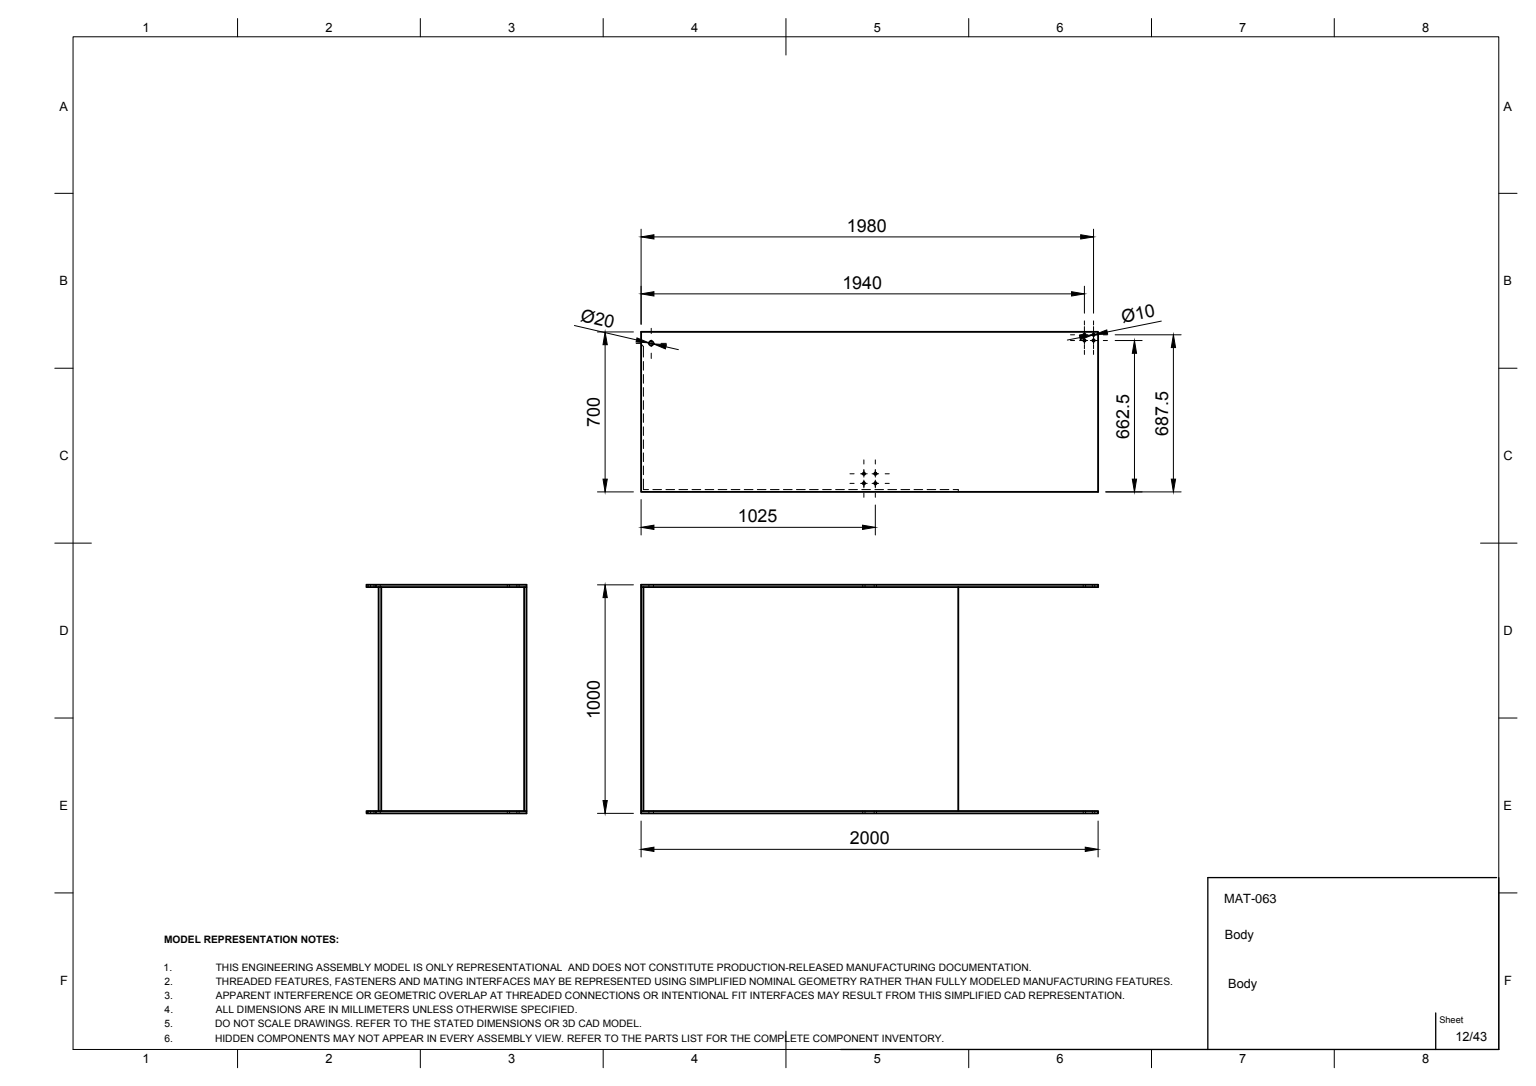
ISO-10303-21;
HEADER;
/* Generated by software containing ST-Developer
 * from STEP Tools, Inc. (www.steptools.com) 
 */

FILE_DESCRIPTION(
/* description */ (''),
/* implementation_level */ '2;1');

FILE_NAME(
/* name */ 'Body.step',
/* time_stamp */ '2026-10-24T09:43:01-07:00',
/* author */ (''),
/* organization */ (''),
/* preprocessor_version */ 'ST-DEVELOPER v20.2',
/* originating_system */ 'Autodesk Translation Framework v15.15.0.0',
/* authorisation */ '');

FILE_SCHEMA (('AUTOMOTIVE_DESIGN { 1 0 10303 214 3 1 1 }'));
ENDSEC;

DATA;
#10=MECHANICAL_DESIGN_GEOMETRIC_PRESENTATION_REPRESENTATION('',(#289),#11112);
#223=SHAPE_REPRESENTATION_RELATIONSHIP('SRR','None',#11247,#256);
#256=ADVANCED_BREP_SHAPE_REPRESENTATION('',(#322),#11092);
#289=STYLED_ITEM('',(#11426),#322);
#322=MANIFOLD_SOLID_BREP('Body',#6026);
#417=FACE_BOUND('',#1348,.T.);
#418=FACE_BOUND('',#1349,.T.);
#419=FACE_BOUND('',#1350,.T.);
#420=FACE_BOUND('',#1351,.T.);
#421=FACE_BOUND('',#1352,.T.);
#422=FACE_BOUND('',#1353,.T.);
#423=FACE_BOUND('',#1354,.T.);
#424=FACE_BOUND('',#1355,.T.);
#425=FACE_BOUND('',#1356,.T.);
#426=FACE_BOUND('',#1358,.T.);
#427=FACE_BOUND('',#1359,.T.);
#428=FACE_BOUND('',#1360,.T.);
#429=FACE_BOUND('',#1361,.T.);
#430=FACE_BOUND('',#1362,.T.);
#431=FACE_BOUND('',#1363,.T.);
#432=FACE_BOUND('',#1364,.T.);
#433=FACE_BOUND('',#1365,.T.);
#434=FACE_BOUND('',#1366,.T.);
#435=FACE_BOUND('',#1385,.T.);
#436=FACE_BOUND('',#1386,.T.);
#437=FACE_BOUND('',#1387,.T.);
#438=FACE_BOUND('',#1388,.T.);
#439=FACE_BOUND('',#1389,.T.);
#440=FACE_BOUND('',#1390,.T.);
#441=FACE_BOUND('',#1391,.T.);
#442=FACE_BOUND('',#1392,.T.);
#443=FACE_BOUND('',#1393,.T.);
#444=FACE_BOUND('',#1395,.T.);
#445=FACE_BOUND('',#1396,.T.);
#446=FACE_BOUND('',#1397,.T.);
#447=FACE_BOUND('',#1398,.T.);
#448=FACE_BOUND('',#1399,.T.);
#449=FACE_BOUND('',#1400,.T.);
#450=FACE_BOUND('',#1401,.T.);
#451=FACE_BOUND('',#1402,.T.);
#452=FACE_BOUND('',#1403,.T.);
#592=PLANE('',#6965);
#593=PLANE('',#6974);
#594=PLANE('',#6991);
#595=PLANE('',#6992);
#596=PLANE('',#6993);
#597=PLANE('',#6994);
#598=PLANE('',#6995);
#599=PLANE('',#6996);
#600=PLANE('',#6997);
#601=PLANE('',#6998);
#602=PLANE('',#6999);
#603=PLANE('',#7000);
#604=PLANE('',#7010);
#605=PLANE('',#7020);
#904=FACE_OUTER_BOUND('',#1346,.T.);
#905=FACE_OUTER_BOUND('',#1347,.T.);
#906=FACE_OUTER_BOUND('',#1357,.T.);
#907=FACE_OUTER_BOUND('',#1367,.T.);
#908=FACE_OUTER_BOUND('',#1368,.T.);
#909=FACE_OUTER_BOUND('',#1369,.T.);
#910=FACE_OUTER_BOUND('',#1370,.T.);
#911=FACE_OUTER_BOUND('',#1371,.T.);
#912=FACE_OUTER_BOUND('',#1372,.T.);
#913=FACE_OUTER_BOUND('',#1373,.T.);
#914=FACE_OUTER_BOUND('',#1374,.T.);
#915=FACE_OUTER_BOUND('',#1375,.T.);
#916=FACE_OUTER_BOUND('',#1376,.T.);
#917=FACE_OUTER_BOUND('',#1377,.T.);
#918=FACE_OUTER_BOUND('',#1378,.T.);
#919=FACE_OUTER_BOUND('',#1379,.T.);
#920=FACE_OUTER_BOUND('',#1380,.T.);
#921=FACE_OUTER_BOUND('',#1381,.T.);
#922=FACE_OUTER_BOUND('',#1382,.T.);
#923=FACE_OUTER_BOUND('',#1383,.T.);
#924=FACE_OUTER_BOUND('',#1384,.T.);
#925=FACE_OUTER_BOUND('',#1394,.T.);
#926=FACE_OUTER_BOUND('',#1404,.T.);
#927=FACE_OUTER_BOUND('',#1405,.T.);
#928=FACE_OUTER_BOUND('',#1406,.T.);
#929=FACE_OUTER_BOUND('',#1407,.T.);
#930=FACE_OUTER_BOUND('',#1408,.T.);
#931=FACE_OUTER_BOUND('',#1409,.T.);
#932=FACE_OUTER_BOUND('',#1410,.T.);
#933=FACE_OUTER_BOUND('',#1411,.T.);
#934=FACE_OUTER_BOUND('',#1412,.T.);
#935=FACE_OUTER_BOUND('',#1413,.T.);
#1346=EDGE_LOOP('',(#4915,#4916,#4917,#4918));
#1347=EDGE_LOOP('',(#4919,#4920,#4921,#4922));
#1348=EDGE_LOOP('',(#4923));
#1349=EDGE_LOOP('',(#4924));
#1350=EDGE_LOOP('',(#4925));
#1351=EDGE_LOOP('',(#4926));
#1352=EDGE_LOOP('',(#4927));
#1353=EDGE_LOOP('',(#4928));
#1354=EDGE_LOOP('',(#4929));
#1355=EDGE_LOOP('',(#4930));
#1356=EDGE_LOOP('',(#4931));
#1357=EDGE_LOOP('',(#4932,#4933,#4934,#4935,#4936,#4937,#4938,#4939));
#1358=EDGE_LOOP('',(#4940));
#1359=EDGE_LOOP('',(#4941));
#1360=EDGE_LOOP('',(#4942));
#1361=EDGE_LOOP('',(#4943));
#1362=EDGE_LOOP('',(#4944));
#1363=EDGE_LOOP('',(#4945));
#1364=EDGE_LOOP('',(#4946));
#1365=EDGE_LOOP('',(#4947));
#1366=EDGE_LOOP('',(#4948));
#1367=EDGE_LOOP('',(#4949,#4950,#4951,#4952));
#1368=EDGE_LOOP('',(#4953,#4954,#4955,#4956));
#1369=EDGE_LOOP('',(#4957,#4958,#4959,#4960));
#1370=EDGE_LOOP('',(#4961,#4962,#4963,#4964));
#1371=EDGE_LOOP('',(#4965,#4966,#4967,#4968));
#1372=EDGE_LOOP('',(#4969,#4970,#4971,#4972));
#1373=EDGE_LOOP('',(#4973,#4974,#4975,#4976));
#1374=EDGE_LOOP('',(#4977,#4978,#4979,#4980));
#1375=EDGE_LOOP('',(#4981,#4982,#4983,#4984,#4985,#4986,#4987,#4988));
#1376=EDGE_LOOP('',(#4989,#4990,#4991,#4992));
#1377=EDGE_LOOP('',(#4993,#4994,#4995,#4996));
#1378=EDGE_LOOP('',(#4997,#4998,#4999,#5000,#5001,#5002,#5003,#5004));
#1379=EDGE_LOOP('',(#5005,#5006,#5007,#5008));
#1380=EDGE_LOOP('',(#5009,#5010,#5011,#5012));
#1381=EDGE_LOOP('',(#5013,#5014,#5015,#5016));
#1382=EDGE_LOOP('',(#5017,#5018,#5019,#5020));
#1383=EDGE_LOOP('',(#5021,#5022,#5023,#5024));
#1384=EDGE_LOOP('',(#5025,#5026,#5027,#5028,#5029,#5030,#5031,#5032));
#1385=EDGE_LOOP('',(#5033));
#1386=EDGE_LOOP('',(#5034));
#1387=EDGE_LOOP('',(#5035));
#1388=EDGE_LOOP('',(#5036));
#1389=EDGE_LOOP('',(#5037));
#1390=EDGE_LOOP('',(#5038));
#1391=EDGE_LOOP('',(#5039));
#1392=EDGE_LOOP('',(#5040));
#1393=EDGE_LOOP('',(#5041));
#1394=EDGE_LOOP('',(#5042,#5043,#5044,#5045));
#1395=EDGE_LOOP('',(#5046));
#1396=EDGE_LOOP('',(#5047));
#1397=EDGE_LOOP('',(#5048));
#1398=EDGE_LOOP('',(#5049));
#1399=EDGE_LOOP('',(#5050));
#1400=EDGE_LOOP('',(#5051));
#1401=EDGE_LOOP('',(#5052));
#1402=EDGE_LOOP('',(#5053));
#1403=EDGE_LOOP('',(#5054));
#1404=EDGE_LOOP('',(#5055,#5056,#5057,#5058));
#1405=EDGE_LOOP('',(#5059,#5060,#5061,#5062));
#1406=EDGE_LOOP('',(#5063,#5064,#5065,#5066));
#1407=EDGE_LOOP('',(#5067,#5068,#5069,#5070));
#1408=EDGE_LOOP('',(#5071,#5072,#5073,#5074));
#1409=EDGE_LOOP('',(#5075,#5076,#5077,#5078));
#1410=EDGE_LOOP('',(#5079,#5080,#5081,#5082));
#1411=EDGE_LOOP('',(#5083,#5084,#5085,#5086));
#1412=EDGE_LOOP('',(#5087,#5088,#5089,#5090));
#1413=EDGE_LOOP('',(#5091,#5092,#5093,#5094));
#1741=LINE('',#10369,#2100);
#1742=LINE('',#10374,#2101);
#1743=LINE('',#10376,#2102);
#1744=LINE('',#10378,#2103);
#1745=LINE('',#10379,#2104);
#1746=LINE('',#10399,#2105);
#1747=LINE('',#10401,#2106);
#1748=LINE('',#10403,#2107);
#1749=LINE('',#10405,#2108);
#1750=LINE('',#10407,#2109);
#1751=LINE('',#10409,#2110);
#1752=LINE('',#10411,#2111);
#1753=LINE('',#10412,#2112);
#1754=LINE('',#10430,#2113);
#1755=LINE('',#10432,#2114);
#1756=LINE('',#10434,#2115);
#1757=LINE('',#10436,#2116);
#1758=LINE('',#10438,#2117);
#1759=LINE('',#10440,#2118);
#1760=LINE('',#10442,#2119);
#1761=LINE('',#10444,#2120);
#1762=LINE('',#10448,#2121);
#1763=LINE('',#10450,#2122);
#1764=LINE('',#10452,#2123);
#1765=LINE('',#10453,#2124);
#1766=LINE('',#10454,#2125);
#1767=LINE('',#10455,#2126);
#1768=LINE('',#10457,#2127);
#1769=LINE('',#10459,#2128);
#1770=LINE('',#10462,#2129);
#1771=LINE('',#10464,#2130);
#1772=LINE('',#10466,#2131);
#1773=LINE('',#10467,#2132);
#1774=LINE('',#10470,#2133);
#1775=LINE('',#10471,#2134);
#1776=LINE('',#10474,#2135);
#1777=LINE('',#10475,#2136);
#1778=LINE('',#10478,#2137);
#1779=LINE('',#10479,#2138);
#1780=LINE('',#10481,#2139);
#1781=LINE('',#10485,#2140);
#1782=LINE('',#10486,#2141);
#1783=LINE('',#10487,#2142);
#1784=LINE('',#10489,#2143);
#1785=LINE('',#10509,#2144);
#1786=LINE('',#10530,#2145);
#1787=LINE('',#10532,#2146);
#1788=LINE('',#10534,#2147);
#1789=LINE('',#10536,#2148);
#1790=LINE('',#10538,#2149);
#1791=LINE('',#10540,#2150);
#1792=LINE('',#10542,#2151);
#1793=LINE('',#10544,#2152);
#1794=LINE('',#10546,#2153);
#2100=VECTOR('',#8557,0.01);
#2101=VECTOR('',#8562,0.01);
#2102=VECTOR('',#8563,0.01);
#2103=VECTOR('',#8564,0.01);
#2104=VECTOR('',#8565,0.01);
#2105=VECTOR('',#8584,0.01);
#2106=VECTOR('',#8585,0.01);
#2107=VECTOR('',#8586,0.01);
#2108=VECTOR('',#8587,0.01);
#2109=VECTOR('',#8588,0.01);
#2110=VECTOR('',#8589,0.01);
#2111=VECTOR('',#8590,0.01);
#2112=VECTOR('',#8591,0.01);
#2113=VECTOR('',#8610,0.00499999999997557);
#2114=VECTOR('',#8613,0.00499999999997558);
#2115=VECTOR('',#8616,0.00500000000000013);
#2116=VECTOR('',#8619,0.005);
#2117=VECTOR('',#8622,0.005);
#2118=VECTOR('',#8625,0.00500000000000013);
#2119=VECTOR('',#8628,0.00499999999997557);
#2120=VECTOR('',#8631,0.00499999999997558);
#2121=VECTOR('',#8634,0.01);
#2122=VECTOR('',#8635,0.01);
#2123=VECTOR('',#8636,0.01);
#2124=VECTOR('',#8637,0.01);
#2125=VECTOR('',#8638,0.01);
#2126=VECTOR('',#8639,0.01);
#2127=VECTOR('',#8642,0.01);
#2128=VECTOR('',#8645,0.01);
#2129=VECTOR('',#8648,0.01);
#2130=VECTOR('',#8649,0.01);
#2131=VECTOR('',#8650,0.01);
#2132=VECTOR('',#8651,0.01);
#2133=VECTOR('',#8654,0.01);
#2134=VECTOR('',#8655,0.01);
#2135=VECTOR('',#8658,0.01);
#2136=VECTOR('',#8659,0.01);
#2137=VECTOR('',#8662,0.01);
#2138=VECTOR('',#8663,0.01);
#2139=VECTOR('',#8666,0.01);
#2140=VECTOR('',#8669,0.01);
#2141=VECTOR('',#8670,0.01);
#2142=VECTOR('',#8671,0.01);
#2143=VECTOR('',#8674,0.01);
#2144=VECTOR('',#8695,0.01);
#2145=VECTOR('',#8718,0.005);
#2146=VECTOR('',#8721,0.005);
#2147=VECTOR('',#8724,0.00500000000000013);
#2148=VECTOR('',#8727,0.005);
#2149=VECTOR('',#8730,0.005);
#2150=VECTOR('',#8733,0.00500000000000013);
#2151=VECTOR('',#8736,0.005);
#2152=VECTOR('',#8739,0.005);
#2153=VECTOR('',#8742,0.01);
#2574=CIRCLE('',#6963,0.01);
#2575=CIRCLE('',#6964,0.01);
#2576=CIRCLE('',#6966,0.00499999999997558);
#2577=CIRCLE('',#6967,0.00499999999997557);
#2578=CIRCLE('',#6968,0.00500000000000013);
#2579=CIRCLE('',#6969,0.005);
#2580=CIRCLE('',#6970,0.005);
#2581=CIRCLE('',#6971,0.00500000000000013);
#2582=CIRCLE('',#6972,0.00499999999997558);
#2583=CIRCLE('',#6973,0.00499999999997557);
#2584=CIRCLE('',#6975,0.00499999999997558);
#2585=CIRCLE('',#6976,0.00499999999997557);
#2586=CIRCLE('',#6977,0.00500000000000013);
#2587=CIRCLE('',#6978,0.005);
#2588=CIRCLE('',#6979,0.005);
#2589=CIRCLE('',#6980,0.00500000000000013);
#2590=CIRCLE('',#6981,0.00499999999997558);
#2591=CIRCLE('',#6982,0.00499999999997557);
#2592=CIRCLE('',#7001,0.01);
#2593=CIRCLE('',#7002,0.005);
#2594=CIRCLE('',#7003,0.005);
#2595=CIRCLE('',#7004,0.00500000000000013);
#2596=CIRCLE('',#7005,0.005);
#2597=CIRCLE('',#7006,0.005);
#2598=CIRCLE('',#7007,0.00500000000000013);
#2599=CIRCLE('',#7008,0.005);
#2600=CIRCLE('',#7009,0.005);
#2601=CIRCLE('',#7011,0.01);
#2602=CIRCLE('',#7012,0.005);
#2603=CIRCLE('',#7013,0.005);
#2604=CIRCLE('',#7014,0.00500000000000013);
#2605=CIRCLE('',#7015,0.005);
#2606=CIRCLE('',#7016,0.005);
#2607=CIRCLE('',#7017,0.00500000000000013);
#2608=CIRCLE('',#7018,0.005);
#2609=CIRCLE('',#7019,0.005);
#2984=VERTEX_POINT('',#10366);
#2985=VERTEX_POINT('',#10368);
#2986=VERTEX_POINT('',#10372);
#2987=VERTEX_POINT('',#10373);
#2988=VERTEX_POINT('',#10375);
#2989=VERTEX_POINT('',#10377);
#2990=VERTEX_POINT('',#10380);
#2991=VERTEX_POINT('',#10382);
#2992=VERTEX_POINT('',#10384);
#2993=VERTEX_POINT('',#10386);
#2994=VERTEX_POINT('',#10388);
#2995=VERTEX_POINT('',#10390);
#2996=VERTEX_POINT('',#10392);
#2997=VERTEX_POINT('',#10394);
#2998=VERTEX_POINT('',#10397);
#2999=VERTEX_POINT('',#10398);
#3000=VERTEX_POINT('',#10400);
#3001=VERTEX_POINT('',#10402);
#3002=VERTEX_POINT('',#10404);
#3003=VERTEX_POINT('',#10406);
#3004=VERTEX_POINT('',#10408);
#3005=VERTEX_POINT('',#10410);
#3006=VERTEX_POINT('',#10413);
#3007=VERTEX_POINT('',#10415);
#3008=VERTEX_POINT('',#10417);
#3009=VERTEX_POINT('',#10419);
#3010=VERTEX_POINT('',#10421);
#3011=VERTEX_POINT('',#10423);
#3012=VERTEX_POINT('',#10425);
#3013=VERTEX_POINT('',#10427);
#3014=VERTEX_POINT('',#10446);
#3015=VERTEX_POINT('',#10447);
#3016=VERTEX_POINT('',#10449);
#3017=VERTEX_POINT('',#10451);
#3018=VERTEX_POINT('',#10461);
#3019=VERTEX_POINT('',#10463);
#3020=VERTEX_POINT('',#10465);
#3021=VERTEX_POINT('',#10469);
#3022=VERTEX_POINT('',#10473);
#3023=VERTEX_POINT('',#10477);
#3024=VERTEX_POINT('',#10483);
#3025=VERTEX_POINT('',#10484);
#3026=VERTEX_POINT('',#10490);
#3027=VERTEX_POINT('',#10492);
#3028=VERTEX_POINT('',#10494);
#3029=VERTEX_POINT('',#10496);
#3030=VERTEX_POINT('',#10498);
#3031=VERTEX_POINT('',#10500);
#3032=VERTEX_POINT('',#10502);
#3033=VERTEX_POINT('',#10504);
#3034=VERTEX_POINT('',#10506);
#3035=VERTEX_POINT('',#10510);
#3036=VERTEX_POINT('',#10512);
#3037=VERTEX_POINT('',#10514);
#3038=VERTEX_POINT('',#10516);
#3039=VERTEX_POINT('',#10518);
#3040=VERTEX_POINT('',#10520);
#3041=VERTEX_POINT('',#10522);
#3042=VERTEX_POINT('',#10524);
#3043=VERTEX_POINT('',#10526);
#3661=EDGE_CURVE('',#2984,#2984,#2574,.T.);
#3662=EDGE_CURVE('',#2984,#2985,#1741,.T.);
#3663=EDGE_CURVE('',#2985,#2985,#2575,.F.);
#3664=EDGE_CURVE('',#2986,#2987,#1742,.T.);
#3665=EDGE_CURVE('',#2988,#2986,#1743,.T.);
#3666=EDGE_CURVE('',#2989,#2988,#1744,.T.);
#3667=EDGE_CURVE('',#2987,#2989,#1745,.T.);
#3668=EDGE_CURVE('',#2990,#2990,#2576,.T.);
#3669=EDGE_CURVE('',#2991,#2991,#2577,.T.);
#3670=EDGE_CURVE('',#2992,#2992,#2578,.F.);
#3671=EDGE_CURVE('',#2993,#2993,#2579,.F.);
#3672=EDGE_CURVE('',#2994,#2994,#2580,.F.);
#3673=EDGE_CURVE('',#2995,#2995,#2581,.F.);
#3674=EDGE_CURVE('',#2996,#2996,#2582,.T.);
#3675=EDGE_CURVE('',#2997,#2997,#2583,.T.);
#3676=EDGE_CURVE('',#2998,#2999,#1746,.T.);
#3677=EDGE_CURVE('',#2999,#3000,#1747,.T.);
#3678=EDGE_CURVE('',#3000,#3001,#1748,.T.);
#3679=EDGE_CURVE('',#3001,#3002,#1749,.T.);
#3680=EDGE_CURVE('',#3002,#3003,#1750,.T.);
#3681=EDGE_CURVE('',#3003,#3004,#1751,.T.);
#3682=EDGE_CURVE('',#3004,#3005,#1752,.T.);
#3683=EDGE_CURVE('',#3005,#2998,#1753,.T.);
#3684=EDGE_CURVE('',#3006,#3006,#2584,.T.);
#3685=EDGE_CURVE('',#3007,#3007,#2585,.T.);
#3686=EDGE_CURVE('',#3008,#3008,#2586,.F.);
#3687=EDGE_CURVE('',#3009,#3009,#2587,.F.);
#3688=EDGE_CURVE('',#3010,#3010,#2588,.F.);
#3689=EDGE_CURVE('',#3011,#3011,#2589,.F.);
#3690=EDGE_CURVE('',#3012,#3012,#2590,.T.);
#3691=EDGE_CURVE('',#3013,#3013,#2591,.T.);
#3692=EDGE_CURVE('',#3013,#2997,#1754,.T.);
#3693=EDGE_CURVE('',#3006,#2996,#1755,.T.);
#3694=EDGE_CURVE('',#2995,#3011,#1756,.T.);
#3695=EDGE_CURVE('',#2994,#3010,#1757,.T.);
#3696=EDGE_CURVE('',#2993,#3009,#1758,.T.);
#3697=EDGE_CURVE('',#2992,#3008,#1759,.T.);
#3698=EDGE_CURVE('',#3007,#2991,#1760,.T.);
#3699=EDGE_CURVE('',#3012,#2990,#1761,.T.);
#3700=EDGE_CURVE('',#3014,#3015,#1762,.T.);
#3701=EDGE_CURVE('',#3016,#3014,#1763,.T.);
#3702=EDGE_CURVE('',#3017,#3016,#1764,.T.);
#3703=EDGE_CURVE('',#3001,#3017,#1765,.T.);
#3704=EDGE_CURVE('',#2988,#3000,#1766,.T.);
#3705=EDGE_CURVE('',#3015,#2986,#1767,.T.);
#3706=EDGE_CURVE('',#2989,#2999,#1768,.T.);
#3707=EDGE_CURVE('',#2987,#2998,#1769,.T.);
#3708=EDGE_CURVE('',#3018,#3005,#1770,.T.);
#3709=EDGE_CURVE('',#3019,#3018,#1771,.T.);
#3710=EDGE_CURVE('',#3020,#3019,#1772,.T.);
#3711=EDGE_CURVE('',#3015,#3020,#1773,.T.);
#3712=EDGE_CURVE('',#3021,#3004,#1774,.T.);
#3713=EDGE_CURVE('',#3018,#3021,#1775,.T.);
#3714=EDGE_CURVE('',#3003,#3022,#1776,.T.);
#3715=EDGE_CURVE('',#3022,#3021,#1777,.T.);
#3716=EDGE_CURVE('',#3002,#3023,#1778,.T.);
#3717=EDGE_CURVE('',#3023,#3022,#1779,.T.);
#3718=EDGE_CURVE('',#3017,#3023,#1780,.T.);
#3719=EDGE_CURVE('',#3024,#3025,#1781,.T.);
#3720=EDGE_CURVE('',#3016,#3024,#1782,.T.);
#3721=EDGE_CURVE('',#3025,#3014,#1783,.T.);
#3722=EDGE_CURVE('',#3019,#3024,#1784,.T.);
#3723=EDGE_CURVE('',#3026,#3026,#2592,.T.);
#3724=EDGE_CURVE('',#3027,#3027,#2593,.T.);
#3725=EDGE_CURVE('',#3028,#3028,#2594,.T.);
#3726=EDGE_CURVE('',#3029,#3029,#2595,.F.);
#3727=EDGE_CURVE('',#3030,#3030,#2596,.F.);
#3728=EDGE_CURVE('',#3031,#3031,#2597,.F.);
#3729=EDGE_CURVE('',#3032,#3032,#2598,.F.);
#3730=EDGE_CURVE('',#3033,#3033,#2599,.T.);
#3731=EDGE_CURVE('',#3034,#3034,#2600,.T.);
#3732=EDGE_CURVE('',#3020,#3025,#1785,.T.);
#3733=EDGE_CURVE('',#3035,#3035,#2601,.T.);
#3734=EDGE_CURVE('',#3036,#3036,#2602,.T.);
#3735=EDGE_CURVE('',#3037,#3037,#2603,.T.);
#3736=EDGE_CURVE('',#3038,#3038,#2604,.F.);
#3737=EDGE_CURVE('',#3039,#3039,#2605,.F.);
#3738=EDGE_CURVE('',#3040,#3040,#2606,.F.);
#3739=EDGE_CURVE('',#3041,#3041,#2607,.F.);
#3740=EDGE_CURVE('',#3042,#3042,#2608,.T.);
#3741=EDGE_CURVE('',#3043,#3043,#2609,.T.);
#3742=EDGE_CURVE('',#3043,#3034,#1786,.T.);
#3743=EDGE_CURVE('',#3036,#3033,#1787,.T.);
#3744=EDGE_CURVE('',#3032,#3041,#1788,.T.);
#3745=EDGE_CURVE('',#3031,#3040,#1789,.T.);
#3746=EDGE_CURVE('',#3030,#3039,#1790,.T.);
#3747=EDGE_CURVE('',#3029,#3038,#1791,.T.);
#3748=EDGE_CURVE('',#3037,#3028,#1792,.T.);
#3749=EDGE_CURVE('',#3042,#3027,#1793,.T.);
#3750=EDGE_CURVE('',#3035,#3026,#1794,.T.);
#4915=ORIENTED_EDGE('',*,*,#3661,.F.);
#4916=ORIENTED_EDGE('',*,*,#3662,.T.);
#4917=ORIENTED_EDGE('',*,*,#3663,.F.);
#4918=ORIENTED_EDGE('',*,*,#3662,.F.);
#4919=ORIENTED_EDGE('',*,*,#3664,.F.);
#4920=ORIENTED_EDGE('',*,*,#3665,.F.);
#4921=ORIENTED_EDGE('',*,*,#3666,.F.);
#4922=ORIENTED_EDGE('',*,*,#3667,.F.);
#4923=ORIENTED_EDGE('',*,*,#3663,.T.);
#4924=ORIENTED_EDGE('',*,*,#3668,.F.);
#4925=ORIENTED_EDGE('',*,*,#3669,.F.);
#4926=ORIENTED_EDGE('',*,*,#3670,.F.);
#4927=ORIENTED_EDGE('',*,*,#3671,.F.);
#4928=ORIENTED_EDGE('',*,*,#3672,.F.);
#4929=ORIENTED_EDGE('',*,*,#3673,.F.);
#4930=ORIENTED_EDGE('',*,*,#3674,.F.);
#4931=ORIENTED_EDGE('',*,*,#3675,.F.);
#4932=ORIENTED_EDGE('',*,*,#3676,.T.);
#4933=ORIENTED_EDGE('',*,*,#3677,.T.);
#4934=ORIENTED_EDGE('',*,*,#3678,.T.);
#4935=ORIENTED_EDGE('',*,*,#3679,.T.);
#4936=ORIENTED_EDGE('',*,*,#3680,.T.);
#4937=ORIENTED_EDGE('',*,*,#3681,.T.);
#4938=ORIENTED_EDGE('',*,*,#3682,.T.);
#4939=ORIENTED_EDGE('',*,*,#3683,.T.);
#4940=ORIENTED_EDGE('',*,*,#3661,.T.);
#4941=ORIENTED_EDGE('',*,*,#3684,.T.);
#4942=ORIENTED_EDGE('',*,*,#3685,.T.);
#4943=ORIENTED_EDGE('',*,*,#3686,.T.);
#4944=ORIENTED_EDGE('',*,*,#3687,.T.);
#4945=ORIENTED_EDGE('',*,*,#3688,.T.);
#4946=ORIENTED_EDGE('',*,*,#3689,.T.);
#4947=ORIENTED_EDGE('',*,*,#3690,.T.);
#4948=ORIENTED_EDGE('',*,*,#3691,.T.);
#4949=ORIENTED_EDGE('',*,*,#3691,.F.);
#4950=ORIENTED_EDGE('',*,*,#3692,.T.);
#4951=ORIENTED_EDGE('',*,*,#3675,.T.);
#4952=ORIENTED_EDGE('',*,*,#3692,.F.);
#4953=ORIENTED_EDGE('',*,*,#3684,.F.);
#4954=ORIENTED_EDGE('',*,*,#3693,.T.);
#4955=ORIENTED_EDGE('',*,*,#3674,.T.);
#4956=ORIENTED_EDGE('',*,*,#3693,.F.);
#4957=ORIENTED_EDGE('',*,*,#3673,.T.);
#4958=ORIENTED_EDGE('',*,*,#3694,.T.);
#4959=ORIENTED_EDGE('',*,*,#3689,.F.);
#4960=ORIENTED_EDGE('',*,*,#3694,.F.);
#4961=ORIENTED_EDGE('',*,*,#3672,.T.);
#4962=ORIENTED_EDGE('',*,*,#3695,.T.);
#4963=ORIENTED_EDGE('',*,*,#3688,.F.);
#4964=ORIENTED_EDGE('',*,*,#3695,.F.);
#4965=ORIENTED_EDGE('',*,*,#3671,.T.);
#4966=ORIENTED_EDGE('',*,*,#3696,.T.);
#4967=ORIENTED_EDGE('',*,*,#3687,.F.);
#4968=ORIENTED_EDGE('',*,*,#3696,.F.);
#4969=ORIENTED_EDGE('',*,*,#3670,.T.);
#4970=ORIENTED_EDGE('',*,*,#3697,.T.);
#4971=ORIENTED_EDGE('',*,*,#3686,.F.);
#4972=ORIENTED_EDGE('',*,*,#3697,.F.);
#4973=ORIENTED_EDGE('',*,*,#3685,.F.);
#4974=ORIENTED_EDGE('',*,*,#3698,.T.);
#4975=ORIENTED_EDGE('',*,*,#3669,.T.);
#4976=ORIENTED_EDGE('',*,*,#3698,.F.);
#4977=ORIENTED_EDGE('',*,*,#3690,.F.);
#4978=ORIENTED_EDGE('',*,*,#3699,.T.);
#4979=ORIENTED_EDGE('',*,*,#3668,.T.);
#4980=ORIENTED_EDGE('',*,*,#3699,.F.);
#4981=ORIENTED_EDGE('',*,*,#3700,.F.);
#4982=ORIENTED_EDGE('',*,*,#3701,.F.);
#4983=ORIENTED_EDGE('',*,*,#3702,.F.);
#4984=ORIENTED_EDGE('',*,*,#3703,.F.);
#4985=ORIENTED_EDGE('',*,*,#3678,.F.);
#4986=ORIENTED_EDGE('',*,*,#3704,.F.);
#4987=ORIENTED_EDGE('',*,*,#3665,.T.);
#4988=ORIENTED_EDGE('',*,*,#3705,.F.);
#4989=ORIENTED_EDGE('',*,*,#3666,.T.);
#4990=ORIENTED_EDGE('',*,*,#3704,.T.);
#4991=ORIENTED_EDGE('',*,*,#3677,.F.);
#4992=ORIENTED_EDGE('',*,*,#3706,.F.);
#4993=ORIENTED_EDGE('',*,*,#3706,.T.);
#4994=ORIENTED_EDGE('',*,*,#3676,.F.);
#4995=ORIENTED_EDGE('',*,*,#3707,.F.);
#4996=ORIENTED_EDGE('',*,*,#3667,.T.);
#4997=ORIENTED_EDGE('',*,*,#3664,.T.);
#4998=ORIENTED_EDGE('',*,*,#3707,.T.);
#4999=ORIENTED_EDGE('',*,*,#3683,.F.);
#5000=ORIENTED_EDGE('',*,*,#3708,.F.);
#5001=ORIENTED_EDGE('',*,*,#3709,.F.);
#5002=ORIENTED_EDGE('',*,*,#3710,.F.);
#5003=ORIENTED_EDGE('',*,*,#3711,.F.);
#5004=ORIENTED_EDGE('',*,*,#3705,.T.);
#5005=ORIENTED_EDGE('',*,*,#3708,.T.);
#5006=ORIENTED_EDGE('',*,*,#3682,.F.);
#5007=ORIENTED_EDGE('',*,*,#3712,.F.);
#5008=ORIENTED_EDGE('',*,*,#3713,.F.);
#5009=ORIENTED_EDGE('',*,*,#3712,.T.);
#5010=ORIENTED_EDGE('',*,*,#3681,.F.);
#5011=ORIENTED_EDGE('',*,*,#3714,.T.);
#5012=ORIENTED_EDGE('',*,*,#3715,.T.);
#5013=ORIENTED_EDGE('',*,*,#3680,.F.);
#5014=ORIENTED_EDGE('',*,*,#3716,.T.);
#5015=ORIENTED_EDGE('',*,*,#3717,.T.);
#5016=ORIENTED_EDGE('',*,*,#3714,.F.);
#5017=ORIENTED_EDGE('',*,*,#3703,.T.);
#5018=ORIENTED_EDGE('',*,*,#3718,.T.);
#5019=ORIENTED_EDGE('',*,*,#3716,.F.);
#5020=ORIENTED_EDGE('',*,*,#3679,.F.);
#5021=ORIENTED_EDGE('',*,*,#3719,.F.);
#5022=ORIENTED_EDGE('',*,*,#3720,.F.);
#5023=ORIENTED_EDGE('',*,*,#3701,.T.);
#5024=ORIENTED_EDGE('',*,*,#3721,.F.);
#5025=ORIENTED_EDGE('',*,*,#3702,.T.);
#5026=ORIENTED_EDGE('',*,*,#3720,.T.);
#5027=ORIENTED_EDGE('',*,*,#3722,.F.);
#5028=ORIENTED_EDGE('',*,*,#3709,.T.);
#5029=ORIENTED_EDGE('',*,*,#3713,.T.);
#5030=ORIENTED_EDGE('',*,*,#3715,.F.);
#5031=ORIENTED_EDGE('',*,*,#3717,.F.);
#5032=ORIENTED_EDGE('',*,*,#3718,.F.);
#5033=ORIENTED_EDGE('',*,*,#3723,.F.);
#5034=ORIENTED_EDGE('',*,*,#3724,.F.);
#5035=ORIENTED_EDGE('',*,*,#3725,.F.);
#5036=ORIENTED_EDGE('',*,*,#3726,.F.);
#5037=ORIENTED_EDGE('',*,*,#3727,.F.);
#5038=ORIENTED_EDGE('',*,*,#3728,.F.);
#5039=ORIENTED_EDGE('',*,*,#3729,.F.);
#5040=ORIENTED_EDGE('',*,*,#3730,.F.);
#5041=ORIENTED_EDGE('',*,*,#3731,.F.);
#5042=ORIENTED_EDGE('',*,*,#3700,.T.);
#5043=ORIENTED_EDGE('',*,*,#3711,.T.);
#5044=ORIENTED_EDGE('',*,*,#3732,.T.);
#5045=ORIENTED_EDGE('',*,*,#3721,.T.);
#5046=ORIENTED_EDGE('',*,*,#3733,.T.);
#5047=ORIENTED_EDGE('',*,*,#3734,.T.);
#5048=ORIENTED_EDGE('',*,*,#3735,.T.);
#5049=ORIENTED_EDGE('',*,*,#3736,.T.);
#5050=ORIENTED_EDGE('',*,*,#3737,.T.);
#5051=ORIENTED_EDGE('',*,*,#3738,.T.);
#5052=ORIENTED_EDGE('',*,*,#3739,.T.);
#5053=ORIENTED_EDGE('',*,*,#3740,.T.);
#5054=ORIENTED_EDGE('',*,*,#3741,.T.);
#5055=ORIENTED_EDGE('',*,*,#3732,.F.);
#5056=ORIENTED_EDGE('',*,*,#3710,.T.);
#5057=ORIENTED_EDGE('',*,*,#3722,.T.);
#5058=ORIENTED_EDGE('',*,*,#3719,.T.);
#5059=ORIENTED_EDGE('',*,*,#3741,.F.);
#5060=ORIENTED_EDGE('',*,*,#3742,.T.);
#5061=ORIENTED_EDGE('',*,*,#3731,.T.);
#5062=ORIENTED_EDGE('',*,*,#3742,.F.);
#5063=ORIENTED_EDGE('',*,*,#3734,.F.);
#5064=ORIENTED_EDGE('',*,*,#3743,.T.);
#5065=ORIENTED_EDGE('',*,*,#3730,.T.);
#5066=ORIENTED_EDGE('',*,*,#3743,.F.);
#5067=ORIENTED_EDGE('',*,*,#3729,.T.);
#5068=ORIENTED_EDGE('',*,*,#3744,.T.);
#5069=ORIENTED_EDGE('',*,*,#3739,.F.);
#5070=ORIENTED_EDGE('',*,*,#3744,.F.);
#5071=ORIENTED_EDGE('',*,*,#3728,.T.);
#5072=ORIENTED_EDGE('',*,*,#3745,.T.);
#5073=ORIENTED_EDGE('',*,*,#3738,.F.);
#5074=ORIENTED_EDGE('',*,*,#3745,.F.);
#5075=ORIENTED_EDGE('',*,*,#3727,.T.);
#5076=ORIENTED_EDGE('',*,*,#3746,.T.);
#5077=ORIENTED_EDGE('',*,*,#3737,.F.);
#5078=ORIENTED_EDGE('',*,*,#3746,.F.);
#5079=ORIENTED_EDGE('',*,*,#3726,.T.);
#5080=ORIENTED_EDGE('',*,*,#3747,.T.);
#5081=ORIENTED_EDGE('',*,*,#3736,.F.);
#5082=ORIENTED_EDGE('',*,*,#3747,.F.);
#5083=ORIENTED_EDGE('',*,*,#3735,.F.);
#5084=ORIENTED_EDGE('',*,*,#3748,.T.);
#5085=ORIENTED_EDGE('',*,*,#3725,.T.);
#5086=ORIENTED_EDGE('',*,*,#3748,.F.);
#5087=ORIENTED_EDGE('',*,*,#3740,.F.);
#5088=ORIENTED_EDGE('',*,*,#3749,.T.);
#5089=ORIENTED_EDGE('',*,*,#3724,.T.);
#5090=ORIENTED_EDGE('',*,*,#3749,.F.);
#5091=ORIENTED_EDGE('',*,*,#3733,.F.);
#5092=ORIENTED_EDGE('',*,*,#3750,.T.);
#5093=ORIENTED_EDGE('',*,*,#3723,.T.);
#5094=ORIENTED_EDGE('',*,*,#3750,.F.);
#5586=CYLINDRICAL_SURFACE('',#6962,0.01);
#5587=CYLINDRICAL_SURFACE('',#6983,0.00499999999997557);
#5588=CYLINDRICAL_SURFACE('',#6984,0.00499999999997558);
#5589=CYLINDRICAL_SURFACE('',#6985,0.00500000000000013);
#5590=CYLINDRICAL_SURFACE('',#6986,0.005);
#5591=CYLINDRICAL_SURFACE('',#6987,0.005);
#5592=CYLINDRICAL_SURFACE('',#6988,0.00500000000000013);
#5593=CYLINDRICAL_SURFACE('',#6989,0.00499999999997557);
#5594=CYLINDRICAL_SURFACE('',#6990,0.00499999999997558);
#5595=CYLINDRICAL_SURFACE('',#7021,0.005);
#5596=CYLINDRICAL_SURFACE('',#7022,0.005);
#5597=CYLINDRICAL_SURFACE('',#7023,0.00500000000000013);
#5598=CYLINDRICAL_SURFACE('',#7024,0.005);
#5599=CYLINDRICAL_SURFACE('',#7025,0.005);
#5600=CYLINDRICAL_SURFACE('',#7026,0.00500000000000013);
#5601=CYLINDRICAL_SURFACE('',#7027,0.005);
#5602=CYLINDRICAL_SURFACE('',#7028,0.005);
#5603=CYLINDRICAL_SURFACE('',#7029,0.01);
#5877=ADVANCED_FACE('',(#904),#5586,.F.);
#5878=ADVANCED_FACE('',(#905,#417,#418,#419,#420,#421,#422,#423,#424,#425),
#592,.F.);
#5879=ADVANCED_FACE('',(#906,#426,#427,#428,#429,#430,#431,#432,#433,#434),
#593,.T.);
#5880=ADVANCED_FACE('',(#907),#5587,.F.);
#5881=ADVANCED_FACE('',(#908),#5588,.F.);
#5882=ADVANCED_FACE('',(#909),#5589,.F.);
#5883=ADVANCED_FACE('',(#910),#5590,.F.);
#5884=ADVANCED_FACE('',(#911),#5591,.F.);
#5885=ADVANCED_FACE('',(#912),#5592,.F.);
#5886=ADVANCED_FACE('',(#913),#5593,.F.);
#5887=ADVANCED_FACE('',(#914),#5594,.F.);
#5888=ADVANCED_FACE('',(#915),#594,.F.);
#5889=ADVANCED_FACE('',(#916),#595,.F.);
#5890=ADVANCED_FACE('',(#917),#596,.F.);
#5891=ADVANCED_FACE('',(#918),#597,.F.);
#5892=ADVANCED_FACE('',(#919),#598,.F.);
#5893=ADVANCED_FACE('',(#920),#599,.T.);
#5894=ADVANCED_FACE('',(#921),#600,.T.);
#5895=ADVANCED_FACE('',(#922),#601,.T.);
#5896=ADVANCED_FACE('',(#923),#602,.F.);
#5897=ADVANCED_FACE('',(#924,#435,#436,#437,#438,#439,#440,#441,#442,#443),
#603,.F.);
#5898=ADVANCED_FACE('',(#925,#444,#445,#446,#447,#448,#449,#450,#451,#452),
#604,.T.);
#5899=ADVANCED_FACE('',(#926),#605,.F.);
#5900=ADVANCED_FACE('',(#927),#5595,.F.);
#5901=ADVANCED_FACE('',(#928),#5596,.F.);
#5902=ADVANCED_FACE('',(#929),#5597,.F.);
#5903=ADVANCED_FACE('',(#930),#5598,.F.);
#5904=ADVANCED_FACE('',(#931),#5599,.F.);
#5905=ADVANCED_FACE('',(#932),#5600,.F.);
#5906=ADVANCED_FACE('',(#933),#5601,.F.);
#5907=ADVANCED_FACE('',(#934),#5602,.F.);
#5908=ADVANCED_FACE('',(#935),#5603,.F.);
#6026=CLOSED_SHELL('',(#5877,#5878,#5879,#5880,#5881,#5882,#5883,#5884,
#5885,#5886,#5887,#5888,#5889,#5890,#5891,#5892,#5893,#5894,#5895,#5896,
#5897,#5898,#5899,#5900,#5901,#5902,#5903,#5904,#5905,#5906,#5907,#5908));
#6961=AXIS2_PLACEMENT_3D('',#10364,#8551,#8552);
#6962=AXIS2_PLACEMENT_3D('',#10365,#8553,#8554);
#6963=AXIS2_PLACEMENT_3D('',#10367,#8555,#8556);
#6964=AXIS2_PLACEMENT_3D('',#10370,#8558,#8559);
#6965=AXIS2_PLACEMENT_3D('',#10371,#8560,#8561);
#6966=AXIS2_PLACEMENT_3D('',#10381,#8566,#8567);
#6967=AXIS2_PLACEMENT_3D('',#10383,#8568,#8569);
#6968=AXIS2_PLACEMENT_3D('',#10385,#8570,#8571);
#6969=AXIS2_PLACEMENT_3D('',#10387,#8572,#8573);
#6970=AXIS2_PLACEMENT_3D('',#10389,#8574,#8575);
#6971=AXIS2_PLACEMENT_3D('',#10391,#8576,#8577);
#6972=AXIS2_PLACEMENT_3D('',#10393,#8578,#8579);
#6973=AXIS2_PLACEMENT_3D('',#10395,#8580,#8581);
#6974=AXIS2_PLACEMENT_3D('',#10396,#8582,#8583);
#6975=AXIS2_PLACEMENT_3D('',#10414,#8592,#8593);
#6976=AXIS2_PLACEMENT_3D('',#10416,#8594,#8595);
#6977=AXIS2_PLACEMENT_3D('',#10418,#8596,#8597);
#6978=AXIS2_PLACEMENT_3D('',#10420,#8598,#8599);
#6979=AXIS2_PLACEMENT_3D('',#10422,#8600,#8601);
#6980=AXIS2_PLACEMENT_3D('',#10424,#8602,#8603);
#6981=AXIS2_PLACEMENT_3D('',#10426,#8604,#8605);
#6982=AXIS2_PLACEMENT_3D('',#10428,#8606,#8607);
#6983=AXIS2_PLACEMENT_3D('',#10429,#8608,#8609);
#6984=AXIS2_PLACEMENT_3D('',#10431,#8611,#8612);
#6985=AXIS2_PLACEMENT_3D('',#10433,#8614,#8615);
#6986=AXIS2_PLACEMENT_3D('',#10435,#8617,#8618);
#6987=AXIS2_PLACEMENT_3D('',#10437,#8620,#8621);
#6988=AXIS2_PLACEMENT_3D('',#10439,#8623,#8624);
#6989=AXIS2_PLACEMENT_3D('',#10441,#8626,#8627);
#6990=AXIS2_PLACEMENT_3D('',#10443,#8629,#8630);
#6991=AXIS2_PLACEMENT_3D('',#10445,#8632,#8633);
#6992=AXIS2_PLACEMENT_3D('',#10456,#8640,#8641);
#6993=AXIS2_PLACEMENT_3D('',#10458,#8643,#8644);
#6994=AXIS2_PLACEMENT_3D('',#10460,#8646,#8647);
#6995=AXIS2_PLACEMENT_3D('',#10468,#8652,#8653);
#6996=AXIS2_PLACEMENT_3D('',#10472,#8656,#8657);
#6997=AXIS2_PLACEMENT_3D('',#10476,#8660,#8661);
#6998=AXIS2_PLACEMENT_3D('',#10480,#8664,#8665);
#6999=AXIS2_PLACEMENT_3D('',#10482,#8667,#8668);
#7000=AXIS2_PLACEMENT_3D('',#10488,#8672,#8673);
#7001=AXIS2_PLACEMENT_3D('',#10491,#8675,#8676);
#7002=AXIS2_PLACEMENT_3D('',#10493,#8677,#8678);
#7003=AXIS2_PLACEMENT_3D('',#10495,#8679,#8680);
#7004=AXIS2_PLACEMENT_3D('',#10497,#8681,#8682);
#7005=AXIS2_PLACEMENT_3D('',#10499,#8683,#8684);
#7006=AXIS2_PLACEMENT_3D('',#10501,#8685,#8686);
#7007=AXIS2_PLACEMENT_3D('',#10503,#8687,#8688);
#7008=AXIS2_PLACEMENT_3D('',#10505,#8689,#8690);
#7009=AXIS2_PLACEMENT_3D('',#10507,#8691,#8692);
#7010=AXIS2_PLACEMENT_3D('',#10508,#8693,#8694);
#7011=AXIS2_PLACEMENT_3D('',#10511,#8696,#8697);
#7012=AXIS2_PLACEMENT_3D('',#10513,#8698,#8699);
#7013=AXIS2_PLACEMENT_3D('',#10515,#8700,#8701);
#7014=AXIS2_PLACEMENT_3D('',#10517,#8702,#8703);
#7015=AXIS2_PLACEMENT_3D('',#10519,#8704,#8705);
#7016=AXIS2_PLACEMENT_3D('',#10521,#8706,#8707);
#7017=AXIS2_PLACEMENT_3D('',#10523,#8708,#8709);
#7018=AXIS2_PLACEMENT_3D('',#10525,#8710,#8711);
#7019=AXIS2_PLACEMENT_3D('',#10527,#8712,#8713);
#7020=AXIS2_PLACEMENT_3D('',#10528,#8714,#8715);
#7021=AXIS2_PLACEMENT_3D('',#10529,#8716,#8717);
#7022=AXIS2_PLACEMENT_3D('',#10531,#8719,#8720);
#7023=AXIS2_PLACEMENT_3D('',#10533,#8722,#8723);
#7024=AXIS2_PLACEMENT_3D('',#10535,#8725,#8726);
#7025=AXIS2_PLACEMENT_3D('',#10537,#8728,#8729);
#7026=AXIS2_PLACEMENT_3D('',#10539,#8731,#8732);
#7027=AXIS2_PLACEMENT_3D('',#10541,#8734,#8735);
#7028=AXIS2_PLACEMENT_3D('',#10543,#8737,#8738);
#7029=AXIS2_PLACEMENT_3D('',#10545,#8740,#8741);
#8551=DIRECTION('axis',(0.,0.,1.));
#8552=DIRECTION('refdir',(1.,0.,0.));
#8553=DIRECTION('center_axis',(1.,0.,0.));
#8554=DIRECTION('ref_axis',(0.,0.,-1.));
#8555=DIRECTION('center_axis',(1.,0.,0.));
#8556=DIRECTION('ref_axis',(0.,0.,-1.));
#8557=DIRECTION('',(1.,0.,0.));
#8558=DIRECTION('center_axis',(1.,0.,0.));
#8559=DIRECTION('ref_axis',(0.,0.,-1.));
#8560=DIRECTION('center_axis',(-1.,0.,0.));
#8561=DIRECTION('ref_axis',(0.,0.,1.));
#8562=DIRECTION('',(0.,0.,1.));
#8563=DIRECTION('',(0.,-1.,0.));
#8564=DIRECTION('',(0.,0.,-1.));
#8565=DIRECTION('',(0.,1.,0.));
#8566=DIRECTION('center_axis',(1.,0.,-2.22044604925031E-14));
#8567=DIRECTION('ref_axis',(-2.22044604925031E-14,0.,-1.));
#8568=DIRECTION('center_axis',(1.,0.,-2.22044604925031E-14));
#8569=DIRECTION('ref_axis',(-2.22044604925031E-14,0.,-1.));
#8570=DIRECTION('center_axis',(-1.,0.,0.));
#8571=DIRECTION('ref_axis',(0.,0.,1.));
#8572=DIRECTION('center_axis',(-1.,0.,0.));
#8573=DIRECTION('ref_axis',(0.,0.,1.));
#8574=DIRECTION('center_axis',(-1.,0.,0.));
#8575=DIRECTION('ref_axis',(0.,0.,1.));
#8576=DIRECTION('center_axis',(-1.,0.,0.));
#8577=DIRECTION('ref_axis',(0.,0.,1.));
#8578=DIRECTION('center_axis',(1.,0.,-2.22044604925031E-14));
#8579=DIRECTION('ref_axis',(-2.22044604925031E-14,0.,-1.));
#8580=DIRECTION('center_axis',(1.,0.,-2.22044604925031E-14));
#8581=DIRECTION('ref_axis',(-2.22044604925031E-14,0.,-1.));
#8582=DIRECTION('center_axis',(-1.,-2.40737135441678E-17,-6.64151273659692E-18));
#8583=DIRECTION('ref_axis',(2.40737135441678E-17,-1.,8.32842834445041E-51));
#8584=DIRECTION('',(0.,1.,0.));
#8585=DIRECTION('',(0.,0.,-1.));
#8586=DIRECTION('',(0.,-1.,0.));
#8587=DIRECTION('',(0.,-0.74983784571108,0.66162164802806));
#8588=DIRECTION('',(0.,-1.,0.));
#8589=DIRECTION('',(0.,0.,1.));
#8590=DIRECTION('',(0.,-1.,0.));
#8591=DIRECTION('',(0.,0.,1.));
#8592=DIRECTION('center_axis',(1.,0.,-2.22044604925031E-14));
#8593=DIRECTION('ref_axis',(-2.22044604925031E-14,0.,-1.));
#8594=DIRECTION('center_axis',(1.,0.,-2.22044604925031E-14));
#8595=DIRECTION('ref_axis',(-2.22044604925031E-14,0.,-1.));
#8596=DIRECTION('center_axis',(-1.,0.,0.));
#8597=DIRECTION('ref_axis',(0.,0.,1.));
#8598=DIRECTION('center_axis',(-1.,0.,0.));
#8599=DIRECTION('ref_axis',(0.,0.,1.));
#8600=DIRECTION('center_axis',(-1.,0.,0.));
#8601=DIRECTION('ref_axis',(0.,0.,1.));
#8602=DIRECTION('center_axis',(-1.,0.,0.));
#8603=DIRECTION('ref_axis',(0.,0.,1.));
#8604=DIRECTION('center_axis',(1.,0.,-2.22044604925031E-14));
#8605=DIRECTION('ref_axis',(-2.22044604925031E-14,0.,-1.));
#8606=DIRECTION('center_axis',(1.,0.,-2.22044604925031E-14));
#8607=DIRECTION('ref_axis',(-2.22044604925031E-14,0.,-1.));
#8608=DIRECTION('center_axis',(1.,0.,-2.22044604925031E-14));
#8609=DIRECTION('ref_axis',(-2.22044604925031E-14,0.,-1.));
#8610=DIRECTION('',(1.,0.,-2.22044604925031E-14));
#8611=DIRECTION('center_axis',(1.,0.,-2.22044604925031E-14));
#8612=DIRECTION('ref_axis',(-2.22044604925031E-14,0.,-1.));
#8613=DIRECTION('',(1.,0.,-2.22044604925031E-14));
#8614=DIRECTION('center_axis',(-1.,0.,0.));
#8615=DIRECTION('ref_axis',(0.,0.,1.));
#8616=DIRECTION('',(-1.,0.,0.));
#8617=DIRECTION('center_axis',(-1.,0.,0.));
#8618=DIRECTION('ref_axis',(0.,0.,1.));
#8619=DIRECTION('',(-1.,0.,0.));
#8620=DIRECTION('center_axis',(-1.,0.,0.));
#8621=DIRECTION('ref_axis',(0.,0.,1.));
#8622=DIRECTION('',(-1.,0.,0.));
#8623=DIRECTION('center_axis',(-1.,0.,0.));
#8624=DIRECTION('ref_axis',(0.,0.,1.));
#8625=DIRECTION('',(-1.,0.,0.));
#8626=DIRECTION('center_axis',(1.,0.,-2.22044604925031E-14));
#8627=DIRECTION('ref_axis',(-2.22044604925031E-14,0.,-1.));
#8628=DIRECTION('',(1.,0.,-2.22044604925031E-14));
#8629=DIRECTION('center_axis',(1.,0.,-2.22044604925031E-14));
#8630=DIRECTION('ref_axis',(-2.22044604925031E-14,0.,-1.));
#8631=DIRECTION('',(1.,0.,-2.22044604925031E-14));
#8632=DIRECTION('center_axis',(0.,0.,1.));
#8633=DIRECTION('ref_axis',(1.,0.,0.));
#8634=DIRECTION('',(0.,-1.,0.));
#8635=DIRECTION('',(-1.,0.,0.));
#8636=DIRECTION('',(0.,1.,0.));
#8637=DIRECTION('',(-1.,0.,0.));
#8638=DIRECTION('',(-1.,0.,0.));
#8639=DIRECTION('',(1.,0.,0.));
#8640=DIRECTION('center_axis',(-7.13714802145194E-16,-1.,3.40997071849065E-18));
#8641=DIRECTION('ref_axis',(1.,-7.13714802145194E-16,0.));
#8642=DIRECTION('',(-1.,0.,0.));
#8643=DIRECTION('center_axis',(0.,0.,-1.));
#8644=DIRECTION('ref_axis',(-1.,0.,0.));
#8645=DIRECTION('',(-1.,0.,0.));
#8646=DIRECTION('center_axis',(-7.13714801545295E-18,1.,-3.40997071849065E-18));
#8647=DIRECTION('ref_axis',(-1.,-7.13714801545295E-18,0.));
#8648=DIRECTION('',(1.,0.,0.));
#8649=DIRECTION('',(0.,0.,-1.));
#8650=DIRECTION('',(1.,0.,0.));
#8651=DIRECTION('',(0.,0.,1.));
#8652=DIRECTION('center_axis',(0.,0.,-1.));
#8653=DIRECTION('ref_axis',(-1.,0.,0.));
#8654=DIRECTION('',(1.,0.,0.));
#8655=DIRECTION('',(0.,1.,0.));
#8656=DIRECTION('center_axis',(1.65076892874297E-17,1.,1.19112403377503E-17));
#8657=DIRECTION('ref_axis',(-1.,1.65076892874297E-17,0.));
#8658=DIRECTION('',(-1.,0.,0.));
#8659=DIRECTION('',(0.,0.,1.));
#8660=DIRECTION('center_axis',(-4.85520273159583E-18,-2.05298137436571E-17,
1.));
#8661=DIRECTION('ref_axis',(0.,-1.,-2.05298137436571E-17));
#8662=DIRECTION('',(-1.,0.,0.));
#8663=DIRECTION('',(0.,-1.,0.));
#8664=DIRECTION('center_axis',(-4.02545654738892E-18,0.661621648028061,
0.74983784571108));
#8665=DIRECTION('ref_axis',(-1.44095358341707E-35,-0.74983784571108,0.661621648028061));
#8666=DIRECTION('',(0.,-0.74983784571111,0.661621648028026));
#8667=DIRECTION('center_axis',(-7.13714801246482E-16,-1.,3.40997071849065E-18));
#8668=DIRECTION('ref_axis',(1.,-7.13714801246482E-16,0.));
#8669=DIRECTION('',(-1.,0.,0.));
#8670=DIRECTION('',(0.,0.,1.));
#8671=DIRECTION('',(0.,0.,-1.));
#8672=DIRECTION('center_axis',(-1.,2.40737135441678E-17,6.64151273659692E-18));
#8673=DIRECTION('ref_axis',(-2.40737135441678E-17,-1.,8.32842834445041E-51));
#8674=DIRECTION('',(0.,1.,0.));
#8675=DIRECTION('center_axis',(1.,0.,0.));
#8676=DIRECTION('ref_axis',(0.,0.,-1.));
#8677=DIRECTION('center_axis',(1.,0.,0.));
#8678=DIRECTION('ref_axis',(0.,0.,-1.));
#8679=DIRECTION('center_axis',(1.,0.,0.));
#8680=DIRECTION('ref_axis',(0.,0.,-1.));
#8681=DIRECTION('center_axis',(-1.,0.,0.));
#8682=DIRECTION('ref_axis',(0.,0.,1.));
#8683=DIRECTION('center_axis',(-1.,0.,0.));
#8684=DIRECTION('ref_axis',(0.,0.,1.));
#8685=DIRECTION('center_axis',(-1.,0.,0.));
#8686=DIRECTION('ref_axis',(0.,0.,1.));
#8687=DIRECTION('center_axis',(-1.,0.,0.));
#8688=DIRECTION('ref_axis',(0.,0.,1.));
#8689=DIRECTION('center_axis',(1.,0.,0.));
#8690=DIRECTION('ref_axis',(0.,0.,-1.));
#8691=DIRECTION('center_axis',(1.,0.,0.));
#8692=DIRECTION('ref_axis',(0.,0.,-1.));
#8693=DIRECTION('center_axis',(-1.,0.,0.));
#8694=DIRECTION('ref_axis',(0.,0.,1.));
#8695=DIRECTION('',(0.,1.,0.));
#8696=DIRECTION('center_axis',(1.,0.,0.));
#8697=DIRECTION('ref_axis',(0.,0.,-1.));
#8698=DIRECTION('center_axis',(1.,0.,0.));
#8699=DIRECTION('ref_axis',(0.,0.,-1.));
#8700=DIRECTION('center_axis',(1.,0.,0.));
#8701=DIRECTION('ref_axis',(0.,0.,-1.));
#8702=DIRECTION('center_axis',(-1.,0.,0.));
#8703=DIRECTION('ref_axis',(0.,0.,1.));
#8704=DIRECTION('center_axis',(-1.,0.,0.));
#8705=DIRECTION('ref_axis',(0.,0.,1.));
#8706=DIRECTION('center_axis',(-1.,0.,0.));
#8707=DIRECTION('ref_axis',(0.,0.,1.));
#8708=DIRECTION('center_axis',(-1.,0.,0.));
#8709=DIRECTION('ref_axis',(0.,0.,1.));
#8710=DIRECTION('center_axis',(1.,0.,0.));
#8711=DIRECTION('ref_axis',(0.,0.,-1.));
#8712=DIRECTION('center_axis',(1.,0.,0.));
#8713=DIRECTION('ref_axis',(0.,0.,-1.));
#8714=DIRECTION('center_axis',(0.,0.,-1.));
#8715=DIRECTION('ref_axis',(-1.,0.,0.));
#8716=DIRECTION('center_axis',(1.,0.,0.));
#8717=DIRECTION('ref_axis',(0.,0.,-1.));
#8718=DIRECTION('',(1.,0.,0.));
#8719=DIRECTION('center_axis',(1.,0.,0.));
#8720=DIRECTION('ref_axis',(0.,0.,-1.));
#8721=DIRECTION('',(1.,0.,0.));
#8722=DIRECTION('center_axis',(-1.,0.,0.));
#8723=DIRECTION('ref_axis',(0.,0.,1.));
#8724=DIRECTION('',(-1.,0.,0.));
#8725=DIRECTION('center_axis',(-1.,0.,0.));
#8726=DIRECTION('ref_axis',(0.,0.,1.));
#8727=DIRECTION('',(-1.,0.,0.));
#8728=DIRECTION('center_axis',(-1.,0.,0.));
#8729=DIRECTION('ref_axis',(0.,0.,1.));
#8730=DIRECTION('',(-1.,0.,0.));
#8731=DIRECTION('center_axis',(-1.,0.,0.));
#8732=DIRECTION('ref_axis',(0.,0.,1.));
#8733=DIRECTION('',(-1.,0.,0.));
#8734=DIRECTION('center_axis',(1.,0.,0.));
#8735=DIRECTION('ref_axis',(0.,0.,-1.));
#8736=DIRECTION('',(1.,0.,0.));
#8737=DIRECTION('center_axis',(1.,0.,0.));
#8738=DIRECTION('ref_axis',(0.,0.,-1.));
#8739=DIRECTION('',(1.,0.,0.));
#8740=DIRECTION('center_axis',(1.,0.,0.));
#8741=DIRECTION('ref_axis',(0.,0.,-1.));
#8742=DIRECTION('',(1.,0.,0.));
#10364=CARTESIAN_POINT('',(0.,0.,0.));
#10365=CARTESIAN_POINT('Origin',(-0.657,0.3,-0.955882353));
#10366=CARTESIAN_POINT('',(0.49,0.3,-0.945882353));
#10367=CARTESIAN_POINT('Origin',(0.49,0.3,-0.955882353));
#10368=CARTESIAN_POINT('',(0.5,0.3,-0.945882353));
#10369=CARTESIAN_POINT('',(-0.657,0.3,-0.945882353));
#10370=CARTESIAN_POINT('Origin',(0.5,0.3,-0.955882353));
#10371=CARTESIAN_POINT('Origin',(0.5,-6.21724893790088E-17,-1.74305014866149E-16));
#10372=CARTESIAN_POINT('',(0.499999999999679,-0.34999999999985,-0.999999999999358));
#10373=CARTESIAN_POINT('',(0.499999999999785,-0.34999999999985,0.999999999999358));
#10374=CARTESIAN_POINT('',(0.5,-0.35,-0.9999999995));
#10375=CARTESIAN_POINT('',(0.499999999999891,0.34999999999985,-0.999999999999358));
#10376=CARTESIAN_POINT('',(0.5,0.349999999825,-1.));
#10377=CARTESIAN_POINT('',(0.499999999999995,0.349999999999663,0.999999999999358));
#10378=CARTESIAN_POINT('',(0.5,0.35,0.9999999995));
#10379=CARTESIAN_POINT('',(0.5,-0.349999999825,1.));
#10380=CARTESIAN_POINT('',(0.5,-0.312833309,0.0299999999999509));
#10381=CARTESIAN_POINT('Origin',(0.5,-0.312833309,0.0249999999999754));
#10382=CARTESIAN_POINT('',(0.5,-0.270944436,-0.0200000000000491));
#10383=CARTESIAN_POINT('Origin',(0.5,-0.270944436,-0.0250000000000247));
#10384=CARTESIAN_POINT('',(0.5,0.3375,0.935));
#10385=CARTESIAN_POINT('Origin',(0.5,0.3375,0.94));
#10386=CARTESIAN_POINT('',(0.5,0.3375,0.975));
#10387=CARTESIAN_POINT('Origin',(0.5,0.3375,0.98));
#10388=CARTESIAN_POINT('',(0.5,0.3125,0.975));
#10389=CARTESIAN_POINT('Origin',(0.5,0.3125,0.98));
#10390=CARTESIAN_POINT('',(0.5,0.3125,0.935));
#10391=CARTESIAN_POINT('Origin',(0.5,0.3125,0.94));
#10392=CARTESIAN_POINT('',(0.5,-0.270944436,0.0299999999999509));
#10393=CARTESIAN_POINT('Origin',(0.5,-0.270944436,0.0249999999999754));
#10394=CARTESIAN_POINT('',(0.5,-0.312833309,-0.0200000000000491));
#10395=CARTESIAN_POINT('Origin',(0.5,-0.312833309,-0.0250000000000247));
#10396=CARTESIAN_POINT('Origin',(0.49,-6.21724893790088E-17,-1.74305014866149E-16));
#10397=CARTESIAN_POINT('',(0.490000000000164,-0.349999999999663,0.999999999999358));
#10398=CARTESIAN_POINT('',(0.490000000000005,0.349999999999663,0.999999999999358));
#10399=CARTESIAN_POINT('',(0.49,-0.349999999825,1.));
#10400=CARTESIAN_POINT('',(0.490000000000109,0.34999999999985,-0.999999999999358));
#10401=CARTESIAN_POINT('',(0.49,0.35,0.9999999995));
#10402=CARTESIAN_POINT('',(0.489999999999999,0.297099674089462,-1.00000000005445));
#10403=CARTESIAN_POINT('',(0.49,0.349999999825,-1.));
#10404=CARTESIAN_POINT('',(0.489999999999528,0.285766341000618,-0.990000000000234));
#10405=CARTESIAN_POINT('',(0.49,0.297099673879244,-0.999999999893451));
#10406=CARTESIAN_POINT('',(0.489999999999528,-0.339999999999815,-0.989999999999458));
#10407=CARTESIAN_POINT('',(0.49,0.285766340955704,-0.99));
#10408=CARTESIAN_POINT('',(0.48999999999979,-0.340000000000108,0.388147024999372));
#10409=CARTESIAN_POINT('',(0.49,-0.34,-0.9899999995));
#10410=CARTESIAN_POINT('',(0.489999999999525,-0.349999999999884,0.388147024999355));
#10411=CARTESIAN_POINT('',(0.49,-0.340000000375,0.388147024999997));
#10412=CARTESIAN_POINT('',(0.49,-0.35,0.38814702475));
#10413=CARTESIAN_POINT('',(0.49,-0.270944436,0.0299999999999512));
#10414=CARTESIAN_POINT('Origin',(0.49,-0.270944436,0.0249999999999756));
#10415=CARTESIAN_POINT('',(0.49,-0.270944436,-0.0200000000000489));
#10416=CARTESIAN_POINT('Origin',(0.49,-0.270944436,-0.0250000000000245));
#10417=CARTESIAN_POINT('',(0.49,0.3375,0.935));
#10418=CARTESIAN_POINT('Origin',(0.49,0.3375,0.94));
#10419=CARTESIAN_POINT('',(0.49,0.3375,0.975));
#10420=CARTESIAN_POINT('Origin',(0.49,0.3375,0.98));
#10421=CARTESIAN_POINT('',(0.49,0.3125,0.975));
#10422=CARTESIAN_POINT('Origin',(0.49,0.3125,0.98));
#10423=CARTESIAN_POINT('',(0.49,0.3125,0.935));
#10424=CARTESIAN_POINT('Origin',(0.49,0.3125,0.94));
#10425=CARTESIAN_POINT('',(0.49,-0.312833309,0.0299999999999512));
#10426=CARTESIAN_POINT('Origin',(0.49,-0.312833309,0.0249999999999756));
#10427=CARTESIAN_POINT('',(0.49,-0.312833309,-0.0200000000000489));
#10428=CARTESIAN_POINT('Origin',(0.49,-0.312833309,-0.0250000000000245));
#10429=CARTESIAN_POINT('Origin',(-0.61,-0.312833309,-0.025));
#10430=CARTESIAN_POINT('',(-0.61,-0.312833309,-0.0200000000000244));
#10431=CARTESIAN_POINT('Origin',(-0.61,-0.270944436,0.025));
#10432=CARTESIAN_POINT('',(-0.61,-0.270944436,0.0299999999999756));
#10433=CARTESIAN_POINT('Origin',(0.51,0.3125,0.94));
#10434=CARTESIAN_POINT('',(0.51,0.3125,0.935));
#10435=CARTESIAN_POINT('Origin',(0.51,0.3125,0.98));
#10436=CARTESIAN_POINT('',(0.51,0.3125,0.975));
#10437=CARTESIAN_POINT('Origin',(0.51,0.3375,0.98));
#10438=CARTESIAN_POINT('',(0.51,0.3375,0.975));
#10439=CARTESIAN_POINT('Origin',(0.51,0.3375,0.94));
#10440=CARTESIAN_POINT('',(0.51,0.3375,0.935));
#10441=CARTESIAN_POINT('Origin',(-0.61,-0.270944436,-0.025));
#10442=CARTESIAN_POINT('',(-0.61,-0.270944436,-0.0200000000000244));
#10443=CARTESIAN_POINT('Origin',(-0.61,-0.312833309,0.025));
#10444=CARTESIAN_POINT('',(-0.61,-0.312833309,0.0299999999999756));
#10445=CARTESIAN_POINT('Origin',(-8.71525074330748E-17,-6.21724893790088E-17,
-1.));
#10446=CARTESIAN_POINT('',(-0.499999999999892,0.349999999999775,-0.999999999999358));
#10447=CARTESIAN_POINT('',(-0.499999999999786,-0.349999999999775,-0.999999999999358));
#10448=CARTESIAN_POINT('',(-0.5,0.349999999825,-1.));
#10449=CARTESIAN_POINT('',(-0.490000000000108,0.349999999999775,-0.999999999999358));
#10450=CARTESIAN_POINT('',(-0.49000000025,0.35,-1.));
#10451=CARTESIAN_POINT('',(-0.489999999999988,0.297099674089289,-1.00000000005438));
#10452=CARTESIAN_POINT('',(-0.49,0.297099674375,-1.));
#10453=CARTESIAN_POINT('',(0.48999999975,0.297099674112451,-1.00000000009922));
#10454=CARTESIAN_POINT('',(0.49999999975,0.35,-1.));
#10455=CARTESIAN_POINT('',(-0.49999999975,-0.35,-1.));
#10456=CARTESIAN_POINT('Origin',(0.495,0.35,1.74305014866149E-16));
#10457=CARTESIAN_POINT('',(0.499999999997498,0.35,1.));
#10458=CARTESIAN_POINT('Origin',(0.495,-6.21724893790088E-17,1.));
#10459=CARTESIAN_POINT('',(0.499999999874375,-0.35,1.));
#10460=CARTESIAN_POINT('Origin',(-1.77635683940025E-17,-0.35,-1.74305014866149E-16));
#10461=CARTESIAN_POINT('',(-0.489999999999788,-0.349999999999849,0.388147024999355));
#10462=CARTESIAN_POINT('',(-0.48999999975,-0.35,0.388147024999997));
#10463=CARTESIAN_POINT('',(-0.490000000000164,-0.349999999999663,0.999999999999358));
#10464=CARTESIAN_POINT('',(-0.49,-0.35,0.9999999995));
#10465=CARTESIAN_POINT('',(-0.499999999999892,-0.349999999999775,0.999999999999358));
#10466=CARTESIAN_POINT('',(-0.49999999975,-0.35,1.));
#10467=CARTESIAN_POINT('',(-0.5,-0.35,-0.9999999995));
#10468=CARTESIAN_POINT('Origin',(6.68909372336657E-17,-0.345,0.388147024999997));
#10469=CARTESIAN_POINT('',(-0.489999999999907,-0.340000000000143,0.388147024999361));
#10470=CARTESIAN_POINT('',(-0.489999999755,-0.34,0.388147024999997));
#10471=CARTESIAN_POINT('',(-0.49,-0.349999999911875,0.388147024999998));
#10472=CARTESIAN_POINT('Origin',(-5.27355936696949E-17,-0.34,-0.3009264875));
#10473=CARTESIAN_POINT('',(-0.489999999999528,-0.339999999999815,-0.989999999999458));
#10474=CARTESIAN_POINT('',(0.489999999755,-0.34,-0.99));
#10475=CARTESIAN_POINT('',(-0.49,-0.34,-0.989999999655463));
#10476=CARTESIAN_POINT('Origin',(-6.68909372336657E-17,-0.0271168294999997,
-0.99));
#10477=CARTESIAN_POINT('',(-0.489999999999528,0.285766341000617,-0.990000000000234));
#10478=CARTESIAN_POINT('',(0.489999999755,0.285766341,-0.99));
#10479=CARTESIAN_POINT('',(-0.49,0.285766340843558,-0.99));
#10480=CARTESIAN_POINT('Origin',(-5.27355936696949E-17,0.2914330075,-0.995));
#10481=CARTESIAN_POINT('',(-0.49,0.297099673997167,-0.9999999999975));
#10482=CARTESIAN_POINT('Origin',(-0.495,0.35,1.74305014866149E-16));
#10483=CARTESIAN_POINT('',(-0.490000000000004,0.349999999999663,0.999999999999358));
#10484=CARTESIAN_POINT('',(-0.499999999999995,0.349999999999663,0.999999999999358));
#10485=CARTESIAN_POINT('',(-0.490000000002499,0.35,1.));
#10486=CARTESIAN_POINT('',(-0.489999999999999,0.35,-0.9999999995));
#10487=CARTESIAN_POINT('',(-0.499999999999999,0.35,0.9999999995));
#10488=CARTESIAN_POINT('Origin',(-0.49,-6.21724893790088E-17,-1.74305014866149E-16));
#10489=CARTESIAN_POINT('',(-0.49,-0.349999999825,1.));
#10490=CARTESIAN_POINT('',(-0.49,0.3,-0.945882353));
#10491=CARTESIAN_POINT('Origin',(-0.49,0.3,-0.955882353));
#10492=CARTESIAN_POINT('',(-0.49,-0.312833309,0.03));
#10493=CARTESIAN_POINT('Origin',(-0.49,-0.312833309,0.025));
#10494=CARTESIAN_POINT('',(-0.49,-0.270944436,-0.02));
#10495=CARTESIAN_POINT('Origin',(-0.49,-0.270944436,-0.025));
#10496=CARTESIAN_POINT('',(-0.49,0.3375,0.935));
#10497=CARTESIAN_POINT('Origin',(-0.49,0.3375,0.94));
#10498=CARTESIAN_POINT('',(-0.49,0.3375,0.975));
#10499=CARTESIAN_POINT('Origin',(-0.49,0.3375,0.98));
#10500=CARTESIAN_POINT('',(-0.49,0.3125,0.975));
#10501=CARTESIAN_POINT('Origin',(-0.49,0.3125,0.98));
#10502=CARTESIAN_POINT('',(-0.49,0.3125,0.935));
#10503=CARTESIAN_POINT('Origin',(-0.49,0.3125,0.94));
#10504=CARTESIAN_POINT('',(-0.49,-0.270944436,0.03));
#10505=CARTESIAN_POINT('Origin',(-0.49,-0.270944436,0.025));
#10506=CARTESIAN_POINT('',(-0.49,-0.312833309,-0.02));
#10507=CARTESIAN_POINT('Origin',(-0.49,-0.312833309,-0.025));
#10508=CARTESIAN_POINT('Origin',(-0.5,-6.21724893790088E-17,-1.74305014866149E-16));
#10509=CARTESIAN_POINT('',(-0.5,-0.349999999825,1.));
#10510=CARTESIAN_POINT('',(-0.5,0.3,-0.945882353));
#10511=CARTESIAN_POINT('Origin',(-0.5,0.3,-0.955882353));
#10512=CARTESIAN_POINT('',(-0.5,-0.270944436,0.03));
#10513=CARTESIAN_POINT('Origin',(-0.5,-0.270944436,0.025));
#10514=CARTESIAN_POINT('',(-0.5,-0.270944436,-0.02));
#10515=CARTESIAN_POINT('Origin',(-0.5,-0.270944436,-0.025));
#10516=CARTESIAN_POINT('',(-0.5,0.3375,0.935));
#10517=CARTESIAN_POINT('Origin',(-0.5,0.3375,0.94));
#10518=CARTESIAN_POINT('',(-0.5,0.3375,0.975));
#10519=CARTESIAN_POINT('Origin',(-0.5,0.3375,0.98));
#10520=CARTESIAN_POINT('',(-0.5,0.3125,0.975));
#10521=CARTESIAN_POINT('Origin',(-0.5,0.3125,0.98));
#10522=CARTESIAN_POINT('',(-0.5,0.3125,0.935));
#10523=CARTESIAN_POINT('Origin',(-0.5,0.3125,0.94));
#10524=CARTESIAN_POINT('',(-0.5,-0.312833309,0.03));
#10525=CARTESIAN_POINT('Origin',(-0.5,-0.312833309,0.025));
#10526=CARTESIAN_POINT('',(-0.5,-0.312833309,-0.02));
#10527=CARTESIAN_POINT('Origin',(-0.5,-0.312833309,-0.025));
#10528=CARTESIAN_POINT('Origin',(-0.495,-6.21724893790088E-17,1.));
#10529=CARTESIAN_POINT('Origin',(-0.61,-0.312833309,-0.025));
#10530=CARTESIAN_POINT('',(-0.61,-0.312833309,-0.02));
#10531=CARTESIAN_POINT('Origin',(-0.61,-0.270944436,0.025));
#10532=CARTESIAN_POINT('',(-0.61,-0.270944436,0.03));
#10533=CARTESIAN_POINT('Origin',(0.51,0.3125,0.94));
#10534=CARTESIAN_POINT('',(0.51,0.3125,0.935));
#10535=CARTESIAN_POINT('Origin',(0.51,0.3125,0.98));
#10536=CARTESIAN_POINT('',(0.51,0.3125,0.975));
#10537=CARTESIAN_POINT('Origin',(0.51,0.3375,0.98));
#10538=CARTESIAN_POINT('',(0.51,0.3375,0.975));
#10539=CARTESIAN_POINT('Origin',(0.51,0.3375,0.94));
#10540=CARTESIAN_POINT('',(0.51,0.3375,0.935));
#10541=CARTESIAN_POINT('Origin',(-0.61,-0.270944436,-0.025));
#10542=CARTESIAN_POINT('',(-0.61,-0.270944436,-0.02));
#10543=CARTESIAN_POINT('Origin',(-0.61,-0.312833309,0.025));
#10544=CARTESIAN_POINT('',(-0.61,-0.312833309,0.03));
#10545=CARTESIAN_POINT('Origin',(-0.657,0.3,-0.955882353));
#10546=CARTESIAN_POINT('',(-0.657,0.3,-0.945882353));
#11053=UNCERTAINTY_MEASURE_WITH_UNIT(LENGTH_MEASURE(1.E-5),#11113,
'DISTANCE_ACCURACY_VALUE',
'Maximum model space distance between geometric entities at asserted c
onnectivities');
#11073=UNCERTAINTY_MEASURE_WITH_UNIT(LENGTH_MEASURE(1.E-5),#11113,
'DISTANCE_ACCURACY_VALUE',
'Maximum model space distance between geometric entities at asserted c
onnectivities');
#11092=(
GEOMETRIC_REPRESENTATION_CONTEXT(3)
GLOBAL_UNCERTAINTY_ASSIGNED_CONTEXT((#11053))
GLOBAL_UNIT_ASSIGNED_CONTEXT((#11113,#11114,#11115))
REPRESENTATION_CONTEXT('','3D')
);
#11112=(
GEOMETRIC_REPRESENTATION_CONTEXT(3)
GLOBAL_UNCERTAINTY_ASSIGNED_CONTEXT((#11073))
GLOBAL_UNIT_ASSIGNED_CONTEXT((#11113,#11114,#11115))
REPRESENTATION_CONTEXT('','3D')
);
#11113=(
LENGTH_UNIT()
NAMED_UNIT(*)
SI_UNIT($,.METRE.)
);
#11114=(
NAMED_UNIT(*)
PLANE_ANGLE_UNIT()
SI_UNIT($,.RADIAN.)
);
#11115=(
NAMED_UNIT(*)
SI_UNIT($,.STERADIAN.)
SOLID_ANGLE_UNIT()
);
#11134=SHAPE_DEFINITION_REPRESENTATION(#11179,#11247);
#11179=PRODUCT_DEFINITION_SHAPE('',$,#11286);
#11247=SHAPE_REPRESENTATION('',(#6961),#11092);
#11267=PRODUCT_DEFINITION_CONTEXT('part definition',#11383,'design');
#11286=PRODUCT_DEFINITION('Body','Body',#11324,#11267);
#11324=PRODUCT_DEFINITION_FORMATION('',$,#11403);
#11383=APPLICATION_CONTEXT(
'Core Data for Automotive Mechanical Design Process');
#11384=PRODUCT_CONTEXT('part definition',#11383,'mechanical');
#11403=PRODUCT('Body','Body',$,(#11384));
#11426=PRESENTATION_STYLE_ASSIGNMENT((#11430));
#11430=SURFACE_STYLE_USAGE(.BOTH.,#11434);
#11434=SURFACE_SIDE_STYLE('',(#11438));
#11438=SURFACE_STYLE_FILL_AREA(#11442);
#11442=FILL_AREA_STYLE('Opaque(202,209,238)',(#11446));
#11446=FILL_AREA_STYLE_COLOUR('Opaque(202,209,238)',#11450);
#11450=COLOUR_RGB('Opaque(202,209,238)',0.792156862745098,0.819607843137255,
0.933333333333333);
ENDSEC;
END-ISO-10303-21;
